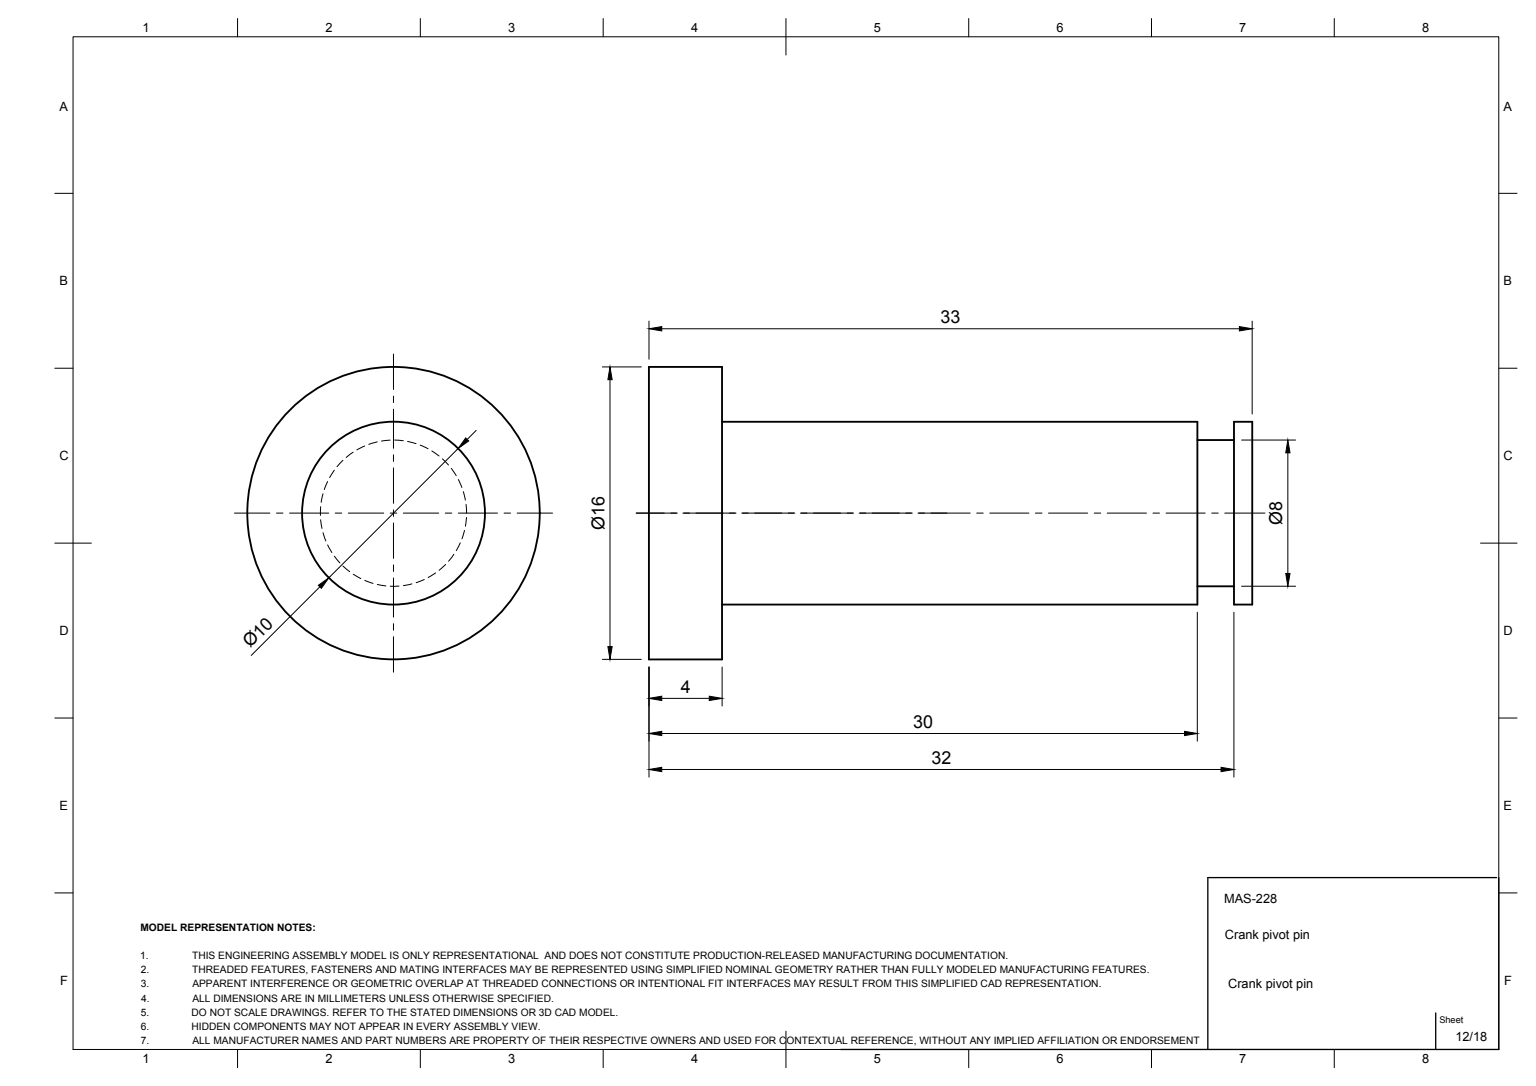
ISO-10303-21;
HEADER;
/* Generated by software containing ST-Developer
 * from STEP Tools, Inc. (www.steptools.com) 
 */

FILE_DESCRIPTION(
/* description */ ('Independent Peaucellier-Lipkin straight-line linkage. Radius arms 100
 mm, inversion-cell links 60 mm, crank radius and fixed-pivot spacing 
32 mm. Inversion constant 6400 mm squared, nominal output straight lin
e X=100 mm. Overhead bearing bridge clears the layered moving links. N
o accuracy or load rating assigned.'),
/* implementation_level */ '2;1');

FILE_NAME(
/* name */ 'Crank pivot pin.step',
/* time_stamp */ '2026-11-09T18:06:16-08:00',
/* author */ (''),
/* organization */ (''),
/* preprocessor_version */ 'ST-DEVELOPER v20.2',
/* originating_system */ 'Autodesk Translation Framework v15.17.0.0',
/* authorisation */ '');

FILE_SCHEMA (('AUTOMOTIVE_DESIGN { 1 0 10303 214 3 1 1 }'));
ENDSEC;

DATA;
#10=MECHANICAL_DESIGN_GEOMETRIC_PRESENTATION_REPRESENTATION('',(#290),#3581);
#256=SHAPE_REPRESENTATION_RELATIONSHIP('SRR','None',#3690,#273);
#273=ADVANCED_BREP_SHAPE_REPRESENTATION('',(#307),#3572);
#290=STYLED_ITEM('',(#3782),#307);
#307=MANIFOLD_SOLID_BREP('Body1',#1876);
#345=FACE_BOUND('',#625,.T.);
#346=FACE_BOUND('',#627,.T.);
#347=FACE_BOUND('',#630,.T.);
#397=PLANE('',#2194);
#398=PLANE('',#2196);
#399=PLANE('',#2200);
#400=PLANE('',#2205);
#401=PLANE('',#2207);
#483=FACE_OUTER_BOUND('',#623,.T.);
#484=FACE_OUTER_BOUND('',#624,.T.);
#485=FACE_OUTER_BOUND('',#626,.T.);
#486=FACE_OUTER_BOUND('',#628,.T.);
#487=FACE_OUTER_BOUND('',#629,.T.);
#488=FACE_OUTER_BOUND('',#631,.T.);
#489=FACE_OUTER_BOUND('',#632,.T.);
#490=FACE_OUTER_BOUND('',#633,.T.);
#491=FACE_OUTER_BOUND('',#634,.T.);
#623=EDGE_LOOP('',(#1550,#1551,#1552,#1553));
#624=EDGE_LOOP('',(#1554));
#625=EDGE_LOOP('',(#1555));
#626=EDGE_LOOP('',(#1556));
#627=EDGE_LOOP('',(#1557));
#628=EDGE_LOOP('',(#1558,#1559,#1560,#1561));
#629=EDGE_LOOP('',(#1562));
#630=EDGE_LOOP('',(#1563));
#631=EDGE_LOOP('',(#1564,#1565,#1566,#1567));
#632=EDGE_LOOP('',(#1568));
#633=EDGE_LOOP('',(#1569,#1570,#1571,#1572));
#634=EDGE_LOOP('',(#1573));
#762=LINE('',#3296,#860);
#763=LINE('',#3307,#861);
#764=LINE('',#3315,#862);
#765=LINE('',#3319,#863);
#860=VECTOR('',#2666,4.);
#861=VECTOR('',#2681,5.);
#862=VECTOR('',#2690,8.);
#863=VECTOR('',#2697,5.);
#941=CIRCLE('',#2192,4.);
#942=CIRCLE('',#2193,4.);
#943=CIRCLE('',#2195,5.);
#944=CIRCLE('',#2197,5.);
#945=CIRCLE('',#2199,5.);
#946=CIRCLE('',#2201,8.);
#947=CIRCLE('',#2202,5.);
#948=CIRCLE('',#2204,8.);
#1067=VERTEX_POINT('',#3293);
#1068=VERTEX_POINT('',#3295);
#1069=VERTEX_POINT('',#3299);
#1070=VERTEX_POINT('',#3302);
#1071=VERTEX_POINT('',#3305);
#1072=VERTEX_POINT('',#3309);
#1073=VERTEX_POINT('',#3311);
#1074=VERTEX_POINT('',#3314);
#1237=EDGE_CURVE('',#1067,#1067,#941,.T.);
#1238=EDGE_CURVE('',#1067,#1068,#762,.T.);
#1239=EDGE_CURVE('',#1068,#1068,#942,.T.);
#1240=EDGE_CURVE('',#1069,#1069,#943,.T.);
#1241=EDGE_CURVE('',#1070,#1070,#944,.T.);
#1242=EDGE_CURVE('',#1071,#1071,#945,.T.);
#1243=EDGE_CURVE('',#1071,#1070,#763,.T.);
#1244=EDGE_CURVE('',#1072,#1072,#946,.T.);
#1245=EDGE_CURVE('',#1073,#1073,#947,.T.);
#1246=EDGE_CURVE('',#1072,#1074,#764,.T.);
#1247=EDGE_CURVE('',#1074,#1074,#948,.T.);
#1248=EDGE_CURVE('',#1069,#1073,#765,.T.);
#1550=ORIENTED_EDGE('',*,*,#1237,.T.);
#1551=ORIENTED_EDGE('',*,*,#1238,.T.);
#1552=ORIENTED_EDGE('',*,*,#1239,.F.);
#1553=ORIENTED_EDGE('',*,*,#1238,.F.);
#1554=ORIENTED_EDGE('',*,*,#1240,.F.);
#1555=ORIENTED_EDGE('',*,*,#1237,.F.);
#1556=ORIENTED_EDGE('',*,*,#1241,.F.);
#1557=ORIENTED_EDGE('',*,*,#1239,.T.);
#1558=ORIENTED_EDGE('',*,*,#1242,.F.);
#1559=ORIENTED_EDGE('',*,*,#1243,.T.);
#1560=ORIENTED_EDGE('',*,*,#1241,.T.);
#1561=ORIENTED_EDGE('',*,*,#1243,.F.);
#1562=ORIENTED_EDGE('',*,*,#1244,.T.);
#1563=ORIENTED_EDGE('',*,*,#1245,.F.);
#1564=ORIENTED_EDGE('',*,*,#1244,.F.);
#1565=ORIENTED_EDGE('',*,*,#1246,.T.);
#1566=ORIENTED_EDGE('',*,*,#1247,.T.);
#1567=ORIENTED_EDGE('',*,*,#1246,.F.);
#1568=ORIENTED_EDGE('',*,*,#1247,.F.);
#1569=ORIENTED_EDGE('',*,*,#1240,.T.);
#1570=ORIENTED_EDGE('',*,*,#1248,.T.);
#1571=ORIENTED_EDGE('',*,*,#1245,.T.);
#1572=ORIENTED_EDGE('',*,*,#1248,.F.);
#1573=ORIENTED_EDGE('',*,*,#1242,.T.);
#1733=CYLINDRICAL_SURFACE('',#2191,4.);
#1734=CYLINDRICAL_SURFACE('',#2198,5.);
#1735=CYLINDRICAL_SURFACE('',#2203,8.);
#1736=CYLINDRICAL_SURFACE('',#2206,5.);
#1815=ADVANCED_FACE('',(#483),#1733,.T.);
#1816=ADVANCED_FACE('',(#484,#345),#397,.F.);
#1817=ADVANCED_FACE('',(#485,#346),#398,.F.);
#1818=ADVANCED_FACE('',(#486),#1734,.T.);
#1819=ADVANCED_FACE('',(#487,#347),#399,.T.);
#1820=ADVANCED_FACE('',(#488),#1735,.T.);
#1821=ADVANCED_FACE('',(#489),#400,.F.);
#1822=ADVANCED_FACE('',(#490),#1736,.T.);
#1823=ADVANCED_FACE('',(#491),#401,.T.);
#1876=CLOSED_SHELL('',(#1815,#1816,#1817,#1818,#1819,#1820,#1821,#1822,
#1823));
#2190=AXIS2_PLACEMENT_3D('',#3291,#2660,#2661);
#2191=AXIS2_PLACEMENT_3D('',#3292,#2662,#2663);
#2192=AXIS2_PLACEMENT_3D('',#3294,#2664,#2665);
#2193=AXIS2_PLACEMENT_3D('',#3297,#2667,#2668);
#2194=AXIS2_PLACEMENT_3D('',#3298,#2669,#2670);
#2195=AXIS2_PLACEMENT_3D('',#3300,#2671,#2672);
#2196=AXIS2_PLACEMENT_3D('',#3301,#2673,#2674);
#2197=AXIS2_PLACEMENT_3D('',#3303,#2675,#2676);
#2198=AXIS2_PLACEMENT_3D('',#3304,#2677,#2678);
#2199=AXIS2_PLACEMENT_3D('',#3306,#2679,#2680);
#2200=AXIS2_PLACEMENT_3D('',#3308,#2682,#2683);
#2201=AXIS2_PLACEMENT_3D('',#3310,#2684,#2685);
#2202=AXIS2_PLACEMENT_3D('',#3312,#2686,#2687);
#2203=AXIS2_PLACEMENT_3D('',#3313,#2688,#2689);
#2204=AXIS2_PLACEMENT_3D('',#3316,#2691,#2692);
#2205=AXIS2_PLACEMENT_3D('',#3317,#2693,#2694);
#2206=AXIS2_PLACEMENT_3D('',#3318,#2695,#2696);
#2207=AXIS2_PLACEMENT_3D('',#3320,#2698,#2699);
#2660=DIRECTION('axis',(0.,0.,1.));
#2661=DIRECTION('refdir',(1.,0.,0.));
#2662=DIRECTION('center_axis',(0.,0.,1.));
#2663=DIRECTION('ref_axis',(1.,0.,0.));
#2664=DIRECTION('center_axis',(0.,0.,1.));
#2665=DIRECTION('ref_axis',(1.,0.,0.));
#2666=DIRECTION('',(0.,0.,1.));
#2667=DIRECTION('center_axis',(0.,0.,1.));
#2668=DIRECTION('ref_axis',(1.,0.,0.));
#2669=DIRECTION('center_axis',(0.,0.,-1.));
#2670=DIRECTION('ref_axis',(-1.,0.,0.));
#2671=DIRECTION('center_axis',(0.,0.,-1.));
#2672=DIRECTION('ref_axis',(1.,0.,0.));
#2673=DIRECTION('center_axis',(0.,0.,1.));
#2674=DIRECTION('ref_axis',(1.,0.,0.));
#2675=DIRECTION('center_axis',(0.,0.,1.));
#2676=DIRECTION('ref_axis',(1.,0.,0.));
#2677=DIRECTION('center_axis',(0.,0.,1.));
#2678=DIRECTION('ref_axis',(1.,0.,0.));
#2679=DIRECTION('center_axis',(0.,0.,1.));
#2680=DIRECTION('ref_axis',(1.,0.,0.));
#2681=DIRECTION('',(0.,0.,-1.));
#2682=DIRECTION('center_axis',(0.,0.,1.));
#2683=DIRECTION('ref_axis',(1.,0.,0.));
#2684=DIRECTION('center_axis',(0.,0.,1.));
#2685=DIRECTION('ref_axis',(1.,0.,0.));
#2686=DIRECTION('center_axis',(0.,0.,1.));
#2687=DIRECTION('ref_axis',(1.,0.,0.));
#2688=DIRECTION('center_axis',(0.,0.,1.));
#2689=DIRECTION('ref_axis',(1.,0.,0.));
#2690=DIRECTION('',(0.,0.,-1.));
#2691=DIRECTION('center_axis',(0.,0.,1.));
#2692=DIRECTION('ref_axis',(1.,0.,0.));
#2693=DIRECTION('center_axis',(0.,0.,1.));
#2694=DIRECTION('ref_axis',(1.,0.,0.));
#2695=DIRECTION('center_axis',(0.,0.,1.));
#2696=DIRECTION('ref_axis',(1.,0.,0.));
#2697=DIRECTION('',(0.,0.,-1.));
#2698=DIRECTION('center_axis',(0.,0.,1.));
#2699=DIRECTION('ref_axis',(1.,0.,0.));
#3291=CARTESIAN_POINT('',(0.,0.,0.));
#3292=CARTESIAN_POINT('Origin',(0.,0.,27.));
#3293=CARTESIAN_POINT('',(-4.,-4.89858719658941E-16,26.));
#3294=CARTESIAN_POINT('Origin',(0.,0.,26.));
#3295=CARTESIAN_POINT('',(-4.,-4.89858719658941E-16,28.));
#3296=CARTESIAN_POINT('',(-4.,-4.89858719658941E-16,27.));
#3297=CARTESIAN_POINT('Origin',(0.,0.,28.));
#3298=CARTESIAN_POINT('Origin',(8.,0.,26.));
#3299=CARTESIAN_POINT('',(-5.,6.12323399573677E-16,26.));
#3300=CARTESIAN_POINT('Origin',(0.,0.,26.));
#3301=CARTESIAN_POINT('Origin',(4.,0.,28.));
#3302=CARTESIAN_POINT('',(-5.,-6.12323399573677E-16,28.));
#3303=CARTESIAN_POINT('Origin',(0.,0.,28.));
#3304=CARTESIAN_POINT('Origin',(0.,0.,0.));
#3305=CARTESIAN_POINT('',(-5.,-6.12323399573677E-16,29.));
#3306=CARTESIAN_POINT('Origin',(0.,0.,29.));
#3307=CARTESIAN_POINT('',(-5.,-6.12323399573677E-16,0.));
#3308=CARTESIAN_POINT('Origin',(0.,0.,0.));
#3309=CARTESIAN_POINT('',(-8.,-9.79717439317883E-16,0.));
#3310=CARTESIAN_POINT('Origin',(0.,0.,0.));
#3311=CARTESIAN_POINT('',(-5.,-6.12323399573677E-16,0.));
#3312=CARTESIAN_POINT('Origin',(0.,0.,0.));
#3313=CARTESIAN_POINT('Origin',(0.,0.,-4.));
#3314=CARTESIAN_POINT('',(-8.,-9.79717439317883E-16,-4.));
#3315=CARTESIAN_POINT('',(-8.,-9.79717439317883E-16,-4.));
#3316=CARTESIAN_POINT('Origin',(0.,0.,-4.));
#3317=CARTESIAN_POINT('Origin',(0.,0.,-4.));
#3318=CARTESIAN_POINT('Origin',(0.,0.,0.));
#3319=CARTESIAN_POINT('',(-5.,-6.12323399573677E-16,0.));
#3320=CARTESIAN_POINT('Origin',(0.,0.,29.));
#3553=UNCERTAINTY_MEASURE_WITH_UNIT(LENGTH_MEASURE(0.01),#3582,
'DISTANCE_ACCURACY_VALUE',
'Maximum model space distance between geometric entities at asserted c
onnectivities');
#3562=UNCERTAINTY_MEASURE_WITH_UNIT(LENGTH_MEASURE(0.01),#3582,
'DISTANCE_ACCURACY_VALUE',
'Maximum model space distance between geometric entities at asserted c
onnectivities');
#3572=(
GEOMETRIC_REPRESENTATION_CONTEXT(3)
GLOBAL_UNCERTAINTY_ASSIGNED_CONTEXT((#3553))
GLOBAL_UNIT_ASSIGNED_CONTEXT((#3582,#3584,#3585))
REPRESENTATION_CONTEXT('','3D')
);
#3581=(
GEOMETRIC_REPRESENTATION_CONTEXT(3)
GLOBAL_UNCERTAINTY_ASSIGNED_CONTEXT((#3562))
GLOBAL_UNIT_ASSIGNED_CONTEXT((#3582,#3584,#3585))
REPRESENTATION_CONTEXT('','3D')
);
#3582=(
LENGTH_UNIT()
NAMED_UNIT(*)
SI_UNIT(.MILLI.,.METRE.)
);
#3584=(
NAMED_UNIT(*)
PLANE_ANGLE_UNIT()
SI_UNIT($,.RADIAN.)
);
#3585=(
NAMED_UNIT(*)
SI_UNIT($,.STERADIAN.)
SOLID_ANGLE_UNIT()
);
#3595=SHAPE_DEFINITION_REPRESENTATION(#3613,#3690);
#3613=PRODUCT_DEFINITION_SHAPE('',$,#3709);
#3690=SHAPE_REPRESENTATION('',(#2190),#3572);
#3699=PRODUCT_DEFINITION_CONTEXT('part definition',#3755,'design');
#3709=PRODUCT_DEFINITION('Crank pivot pin','Crank pivot pin',#3727,#3699);
#3727=PRODUCT_DEFINITION_FORMATION('',$,#3766);
#3755=APPLICATION_CONTEXT(
'Core Data for Automotive Mechanical Design Process');
#3756=PRODUCT_CONTEXT('part definition',#3755,'mechanical');
#3766=PRODUCT('Crank pivot pin','Crank pivot pin',$,(#3756));
#3782=PRESENTATION_STYLE_ASSIGNMENT((#3795));
#3795=SURFACE_STYLE_USAGE(.BOTH.,#3808);
#3808=SURFACE_SIDE_STYLE('',(#3821));
#3821=SURFACE_STYLE_FILL_AREA(#3834);
#3834=FILL_AREA_STYLE('Pivot gray',(#3847));
#3847=FILL_AREA_STYLE_COLOUR('Pivot gray',#3860);
#3860=COLOUR_RGB('Pivot gray',0.407843137254902,0.447058823529412,0.498039215686275);
ENDSEC;
END-ISO-10303-21;
